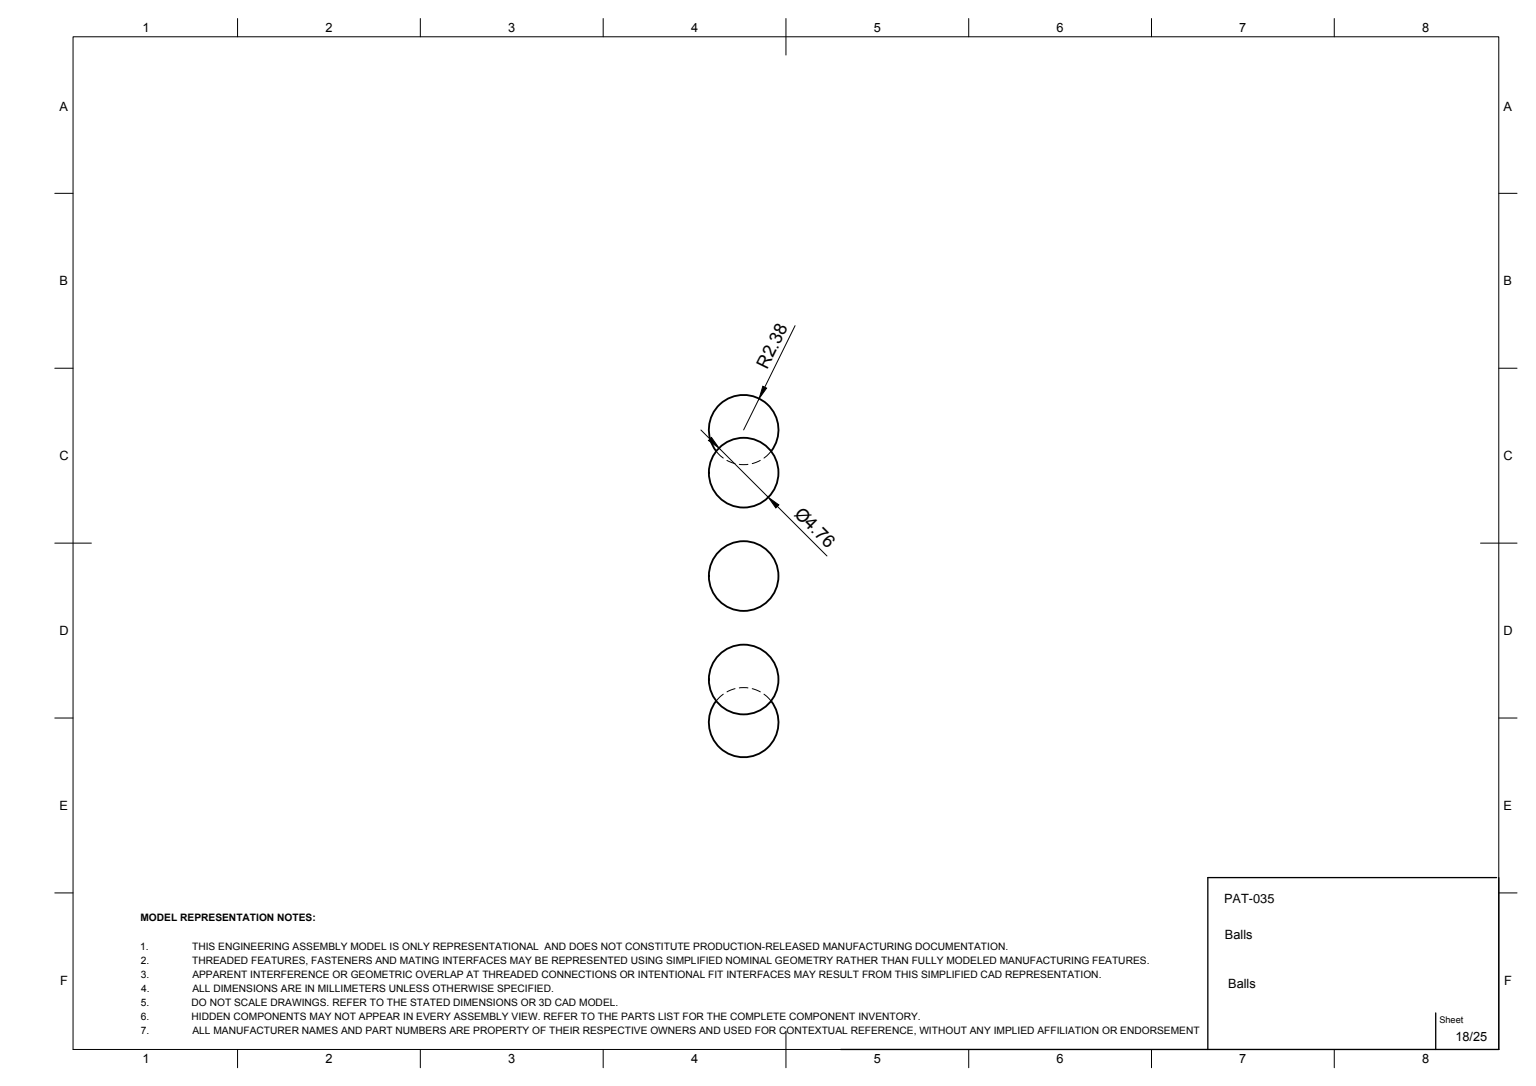
ISO-10303-21;
HEADER;
/* Generated by software containing ST-Developer
 * from STEP Tools, Inc. (www.steptools.com) 
 */

FILE_DESCRIPTION(
/* description */ ('Five-roller gravity conveyor'),
/* implementation_level */ '2;1');

FILE_NAME(
/* name */ 'Balls.step',
/* time_stamp */ '2026-10-29T15:36:43-07:00',
/* author */ (''),
/* organization */ (''),
/* preprocessor_version */ 'ST-DEVELOPER v20.2',
/* originating_system */ 'Autodesk Translation Framework v15.17.0.0',
/* authorisation */ '');

FILE_SCHEMA (('AUTOMOTIVE_DESIGN { 1 0 10303 214 3 1 1 }'));
ENDSEC;

DATA;
#10=MECHANICAL_DESIGN_GEOMETRIC_PRESENTATION_REPRESENTATION('',(#320,#321,#322,#323,#324,#325,#326,#327),#7806);
#241=SPHERICAL_SURFACE('',#4660,0.23815);
#242=SPHERICAL_SURFACE('',#4662,0.23815);
#243=SPHERICAL_SURFACE('',#4664,0.23815);
#244=SPHERICAL_SURFACE('',#4666,0.23815);
#245=SPHERICAL_SURFACE('',#4668,0.23815);
#246=SPHERICAL_SURFACE('',#4670,0.23815);
#247=SPHERICAL_SURFACE('',#4672,0.23815);
#248=SPHERICAL_SURFACE('',#4674,0.23815);
#284=SHAPE_REPRESENTATION_RELATIONSHIP('SRR','None',#7922,#302);
#302=ADVANCED_BREP_SHAPE_REPRESENTATION('',(#345,#346,#347,#348,#349,#350,
#351,#352),#7795);
#320=STYLED_ITEM('',(#8091),#345);
#321=STYLED_ITEM('',(#8091),#346);
#322=STYLED_ITEM('',(#8091),#347);
#323=STYLED_ITEM('',(#8091),#348);
#324=STYLED_ITEM('',(#8091),#349);
#325=STYLED_ITEM('',(#8091),#350);
#326=STYLED_ITEM('',(#8091),#351);
#327=STYLED_ITEM('',(#8091),#352);
#345=MANIFOLD_SOLID_BREP('Body1',#4208);
#346=MANIFOLD_SOLID_BREP('Body2',#4209);
#347=MANIFOLD_SOLID_BREP('Body3',#4210);
#348=MANIFOLD_SOLID_BREP('Body4',#4211);
#349=MANIFOLD_SOLID_BREP('Body5',#4212);
#350=MANIFOLD_SOLID_BREP('Body6',#4213);
#351=MANIFOLD_SOLID_BREP('Body7',#4214);
#352=MANIFOLD_SOLID_BREP('Body8',#4215);
#494=CIRCLE('',#4661,0.23815);
#495=CIRCLE('',#4663,0.23815);
#496=CIRCLE('',#4665,0.23815);
#497=CIRCLE('',#4667,0.23815);
#498=CIRCLE('',#4669,0.23815);
#499=CIRCLE('',#4671,0.23815);
#500=CIRCLE('',#4673,0.23815);
#501=CIRCLE('',#4675,0.23815);
#798=FACE_OUTER_BOUND('',#1054,.T.);
#799=FACE_OUTER_BOUND('',#1055,.T.);
#800=FACE_OUTER_BOUND('',#1056,.T.);
#801=FACE_OUTER_BOUND('',#1057,.T.);
#802=FACE_OUTER_BOUND('',#1058,.T.);
#803=FACE_OUTER_BOUND('',#1059,.T.);
#804=FACE_OUTER_BOUND('',#1060,.T.);
#805=FACE_OUTER_BOUND('',#1061,.T.);
#1054=EDGE_LOOP('',(#3484,#3485));
#1055=EDGE_LOOP('',(#3486,#3487));
#1056=EDGE_LOOP('',(#3488,#3489));
#1057=EDGE_LOOP('',(#3490,#3491));
#1058=EDGE_LOOP('',(#3492,#3493));
#1059=EDGE_LOOP('',(#3494,#3495));
#1060=EDGE_LOOP('',(#3496,#3497));
#1061=EDGE_LOOP('',(#3498,#3499));
#2098=VERTEX_POINT('',#6982);
#2099=VERTEX_POINT('',#6983);
#2100=VERTEX_POINT('',#6986);
#2101=VERTEX_POINT('',#6987);
#2102=VERTEX_POINT('',#6990);
#2103=VERTEX_POINT('',#6991);
#2104=VERTEX_POINT('',#6994);
#2105=VERTEX_POINT('',#6995);
#2106=VERTEX_POINT('',#6998);
#2107=VERTEX_POINT('',#6999);
#2108=VERTEX_POINT('',#7002);
#2109=VERTEX_POINT('',#7003);
#2110=VERTEX_POINT('',#7006);
#2111=VERTEX_POINT('',#7007);
#2112=VERTEX_POINT('',#7010);
#2113=VERTEX_POINT('',#7011);
#2585=EDGE_CURVE('',#2098,#2099,#494,.T.);
#2586=EDGE_CURVE('',#2100,#2101,#495,.T.);
#2587=EDGE_CURVE('',#2102,#2103,#496,.T.);
#2588=EDGE_CURVE('',#2104,#2105,#497,.T.);
#2589=EDGE_CURVE('',#2106,#2107,#498,.T.);
#2590=EDGE_CURVE('',#2108,#2109,#499,.T.);
#2591=EDGE_CURVE('',#2110,#2111,#500,.T.);
#2592=EDGE_CURVE('',#2112,#2113,#501,.T.);
#3484=ORIENTED_EDGE('',*,*,#2585,.T.);
#3485=ORIENTED_EDGE('',*,*,#2585,.F.);
#3486=ORIENTED_EDGE('',*,*,#2586,.T.);
#3487=ORIENTED_EDGE('',*,*,#2586,.F.);
#3488=ORIENTED_EDGE('',*,*,#2587,.T.);
#3489=ORIENTED_EDGE('',*,*,#2587,.F.);
#3490=ORIENTED_EDGE('',*,*,#2588,.T.);
#3491=ORIENTED_EDGE('',*,*,#2588,.F.);
#3492=ORIENTED_EDGE('',*,*,#2589,.T.);
#3493=ORIENTED_EDGE('',*,*,#2589,.F.);
#3494=ORIENTED_EDGE('',*,*,#2590,.T.);
#3495=ORIENTED_EDGE('',*,*,#2590,.F.);
#3496=ORIENTED_EDGE('',*,*,#2591,.T.);
#3497=ORIENTED_EDGE('',*,*,#2591,.F.);
#3498=ORIENTED_EDGE('',*,*,#2592,.T.);
#3499=ORIENTED_EDGE('',*,*,#2592,.F.);
#4113=ADVANCED_FACE('',(#798),#241,.T.);
#4114=ADVANCED_FACE('',(#799),#242,.T.);
#4115=ADVANCED_FACE('',(#800),#243,.T.);
#4116=ADVANCED_FACE('',(#801),#244,.T.);
#4117=ADVANCED_FACE('',(#802),#245,.T.);
#4118=ADVANCED_FACE('',(#803),#246,.T.);
#4119=ADVANCED_FACE('',(#804),#247,.T.);
#4120=ADVANCED_FACE('',(#805),#248,.T.);
#4208=CLOSED_SHELL('',(#4113));
#4209=CLOSED_SHELL('',(#4114));
#4210=CLOSED_SHELL('',(#4115));
#4211=CLOSED_SHELL('',(#4116));
#4212=CLOSED_SHELL('',(#4117));
#4213=CLOSED_SHELL('',(#4118));
#4214=CLOSED_SHELL('',(#4119));
#4215=CLOSED_SHELL('',(#4120));
#4659=AXIS2_PLACEMENT_3D('',#6980,#5665,#5666);
#4660=AXIS2_PLACEMENT_3D('',#6981,#5667,#5668);
#4661=AXIS2_PLACEMENT_3D('',#6984,#5669,#5670);
#4662=AXIS2_PLACEMENT_3D('',#6985,#5671,#5672);
#4663=AXIS2_PLACEMENT_3D('',#6988,#5673,#5674);
#4664=AXIS2_PLACEMENT_3D('',#6989,#5675,#5676);
#4665=AXIS2_PLACEMENT_3D('',#6992,#5677,#5678);
#4666=AXIS2_PLACEMENT_3D('',#6993,#5679,#5680);
#4667=AXIS2_PLACEMENT_3D('',#6996,#5681,#5682);
#4668=AXIS2_PLACEMENT_3D('',#6997,#5683,#5684);
#4669=AXIS2_PLACEMENT_3D('',#7000,#5685,#5686);
#4670=AXIS2_PLACEMENT_3D('',#7001,#5687,#5688);
#4671=AXIS2_PLACEMENT_3D('',#7004,#5689,#5690);
#4672=AXIS2_PLACEMENT_3D('',#7005,#5691,#5692);
#4673=AXIS2_PLACEMENT_3D('',#7008,#5693,#5694);
#4674=AXIS2_PLACEMENT_3D('',#7009,#5695,#5696);
#4675=AXIS2_PLACEMENT_3D('',#7012,#5697,#5698);
#5665=DIRECTION('axis',(0.,0.,1.));
#5666=DIRECTION('refdir',(1.,0.,0.));
#5667=DIRECTION('center_axis',(0.,0.,1.));
#5668=DIRECTION('ref_axis',(1.,0.,0.));
#5669=DIRECTION('center_axis',(1.22464679914735E-16,-1.,0.));
#5670=DIRECTION('ref_axis',(-1.,-1.22464679914735E-16,0.));
#5671=DIRECTION('center_axis',(0.707106781186548,0.,0.707106781186548));
#5672=DIRECTION('ref_axis',(0.707106781186548,0.,-0.707106781186548));
#5673=DIRECTION('center_axis',(8.65956056235494E-17,-1.,-8.65956056235493E-17));
#5674=DIRECTION('ref_axis',(-0.707106781186547,-1.22464679914735E-16,0.707106781186547));
#5675=DIRECTION('center_axis',(1.,0.,0.));
#5676=DIRECTION('ref_axis',(6.12323399573676E-17,0.,-1.));
#5677=DIRECTION('center_axis',(7.49879891330929E-33,-1.,-1.22464679914735E-16));
#5678=DIRECTION('ref_axis',(-6.12323399573676E-17,-1.22464679914735E-16,
1.));
#5679=DIRECTION('center_axis',(0.707106781186548,0.,-0.707106781186548));
#5680=DIRECTION('ref_axis',(-0.707106781186548,0.,-0.707106781186548));
#5681=DIRECTION('center_axis',(-8.65956056235493E-17,-1.,-8.65956056235494E-17));
#5682=DIRECTION('ref_axis',(0.707106781186547,-1.22464679914735E-16,0.707106781186547));
#5683=DIRECTION('center_axis',(0.,0.,-1.));
#5684=DIRECTION('ref_axis',(-1.,0.,-1.22464679914735E-16));
#5685=DIRECTION('center_axis',(-1.22464679914735E-16,-1.,-1.49975978266186E-32));
#5686=DIRECTION('ref_axis',(1.,-1.22464679914735E-16,1.22464679914735E-16));
#5687=DIRECTION('center_axis',(-0.707106781186547,0.,-0.707106781186548));
#5688=DIRECTION('ref_axis',(-0.707106781186548,0.,0.707106781186547));
#5689=DIRECTION('center_axis',(-8.65956056235493E-17,-1.,8.65956056235493E-17));
#5690=DIRECTION('ref_axis',(0.707106781186548,-1.22464679914735E-16,-0.707106781186547));
#5691=DIRECTION('center_axis',(-1.,0.,0.));
#5692=DIRECTION('ref_axis',(-1.83697019872103E-16,0.,1.));
#5693=DIRECTION('center_axis',(-2.24963967399279E-32,-1.,1.22464679914735E-16));
#5694=DIRECTION('ref_axis',(1.83697019872103E-16,-1.22464679914735E-16,
-1.));
#5695=DIRECTION('center_axis',(-0.707106781186548,0.,0.707106781186548));
#5696=DIRECTION('ref_axis',(0.707106781186547,0.,0.707106781186548));
#5697=DIRECTION('center_axis',(8.65956056235493E-17,-1.,8.65956056235493E-17));
#5698=DIRECTION('ref_axis',(-0.707106781186547,-1.22464679914735E-16,-0.707106781186548));
#6980=CARTESIAN_POINT('',(0.,0.,0.));
#6981=CARTESIAN_POINT('Origin',(1.,0.,0.));
#6982=CARTESIAN_POINT('',(1.,-1.78583896120461E-33,0.23815));
#6983=CARTESIAN_POINT('',(1.,-1.78583896120461E-33,-0.23815));
#6984=CARTESIAN_POINT('Origin',(1.,0.,0.));
#6985=CARTESIAN_POINT('Origin',(0.707106781186548,0.,-0.707106781186547));
#6986=CARTESIAN_POINT('',(0.875504261126124,-1.78583896120461E-33,-0.538709301246971));
#6987=CARTESIAN_POINT('',(0.538709301246971,-1.78583896120461E-33,-0.875504261126124));
#6988=CARTESIAN_POINT('Origin',(0.707106781186548,0.,-0.707106781186547));
#6989=CARTESIAN_POINT('Origin',(6.12323399573677E-17,0.,-1.));
#6990=CARTESIAN_POINT('',(0.23815,-1.78583896120461E-33,-1.));
#6991=CARTESIAN_POINT('',(-0.23815,-1.78583896120461E-33,-1.));
#6992=CARTESIAN_POINT('Origin',(6.12323399573677E-17,0.,-1.));
#6993=CARTESIAN_POINT('Origin',(-0.707106781186547,0.,-0.707106781186548));
#6994=CARTESIAN_POINT('',(-0.538709301246971,-1.78583896120461E-33,-0.875504261126124));
#6995=CARTESIAN_POINT('',(-0.875504261126124,-1.78583896120461E-33,-0.538709301246971));
#6996=CARTESIAN_POINT('Origin',(-0.707106781186547,0.,-0.707106781186548));
#6997=CARTESIAN_POINT('Origin',(-1.,0.,-1.22464679914735E-16));
#6998=CARTESIAN_POINT('',(-1.,-1.78583896120461E-33,-0.23815));
#6999=CARTESIAN_POINT('',(-1.,-1.78583896120461E-33,0.23815));
#7000=CARTESIAN_POINT('Origin',(-1.,0.,-1.22464679914735E-16));
#7001=CARTESIAN_POINT('Origin',(-0.707106781186548,0.,0.707106781186547));
#7002=CARTESIAN_POINT('',(-0.875504261126124,-7.94881478324376E-33,0.538709301246971));
#7003=CARTESIAN_POINT('',(-0.538709301246971,4.37713686083455E-33,0.875504261126124));
#7004=CARTESIAN_POINT('Origin',(-0.707106781186548,0.,0.707106781186547));
#7005=CARTESIAN_POINT('Origin',(-1.83697019872103E-16,0.,1.));
#7006=CARTESIAN_POINT('',(-0.23815,-1.78583896120461E-33,1.));
#7007=CARTESIAN_POINT('',(0.23815,-1.78583896120461E-33,1.));
#7008=CARTESIAN_POINT('Origin',(-1.83697019872103E-16,0.,1.));
#7009=CARTESIAN_POINT('Origin',(0.707106781186547,0.,0.707106781186548));
#7010=CARTESIAN_POINT('',(0.538709301246971,-4.86732687222419E-33,0.875504261126124));
#7011=CARTESIAN_POINT('',(0.875504261126124,1.29564894981497E-33,0.538709301246971));
#7012=CARTESIAN_POINT('Origin',(0.707106781186547,0.,0.707106781186548));
#7771=UNCERTAINTY_MEASURE_WITH_UNIT(LENGTH_MEASURE(0.001),#7807,
'DISTANCE_ACCURACY_VALUE',
'Maximum model space distance between geometric entities at asserted c
onnectivities');
#7782=UNCERTAINTY_MEASURE_WITH_UNIT(LENGTH_MEASURE(0.001),#7807,
'DISTANCE_ACCURACY_VALUE',
'Maximum model space distance between geometric entities at asserted c
onnectivities');
#7795=(
GEOMETRIC_REPRESENTATION_CONTEXT(3)
GLOBAL_UNCERTAINTY_ASSIGNED_CONTEXT((#7771))
GLOBAL_UNIT_ASSIGNED_CONTEXT((#7807,#7809,#7810))
REPRESENTATION_CONTEXT('','3D')
);
#7806=(
GEOMETRIC_REPRESENTATION_CONTEXT(3)
GLOBAL_UNCERTAINTY_ASSIGNED_CONTEXT((#7782))
GLOBAL_UNIT_ASSIGNED_CONTEXT((#7807,#7809,#7810))
REPRESENTATION_CONTEXT('','3D')
);
#7807=(
LENGTH_UNIT()
NAMED_UNIT(*)
SI_UNIT(.CENTI.,.METRE.)
);
#7809=(
NAMED_UNIT(*)
PLANE_ANGLE_UNIT()
SI_UNIT($,.RADIAN.)
);
#7810=(
NAMED_UNIT(*)
SI_UNIT($,.STERADIAN.)
SOLID_ANGLE_UNIT()
);
#7823=SHAPE_DEFINITION_REPRESENTATION(#7846,#7922);
#7846=PRODUCT_DEFINITION_SHAPE('',$,#7946);
#7922=SHAPE_REPRESENTATION('',(#4659),#7795);
#7933=PRODUCT_DEFINITION_CONTEXT('part definition',#8004,'design');
#7946=PRODUCT_DEFINITION('Balls','Balls',#7969,#7933);
#7969=PRODUCT_DEFINITION_FORMATION('',$,#8018);
#8004=APPLICATION_CONTEXT(
'Core Data for Automotive Mechanical Design Process');
#8005=PRODUCT_CONTEXT('part definition',#8004,'mechanical');
#8018=PRODUCT('Balls','Balls','Balls',(#8005));
#8085=COLOUR_RGB('Grey',0.48,0.52,0.57);
#8086=FILL_AREA_STYLE_COLOUR('',#8085);
#8087=FILL_AREA_STYLE('',(#8086));
#8088=SURFACE_STYLE_FILL_AREA(#8087);
#8089=SURFACE_SIDE_STYLE('',(#8088));
#8090=SURFACE_STYLE_USAGE(.BOTH.,#8089);
#8091=PRESENTATION_STYLE_ASSIGNMENT((#8090));
ENDSEC;
END-ISO-10303-21;
